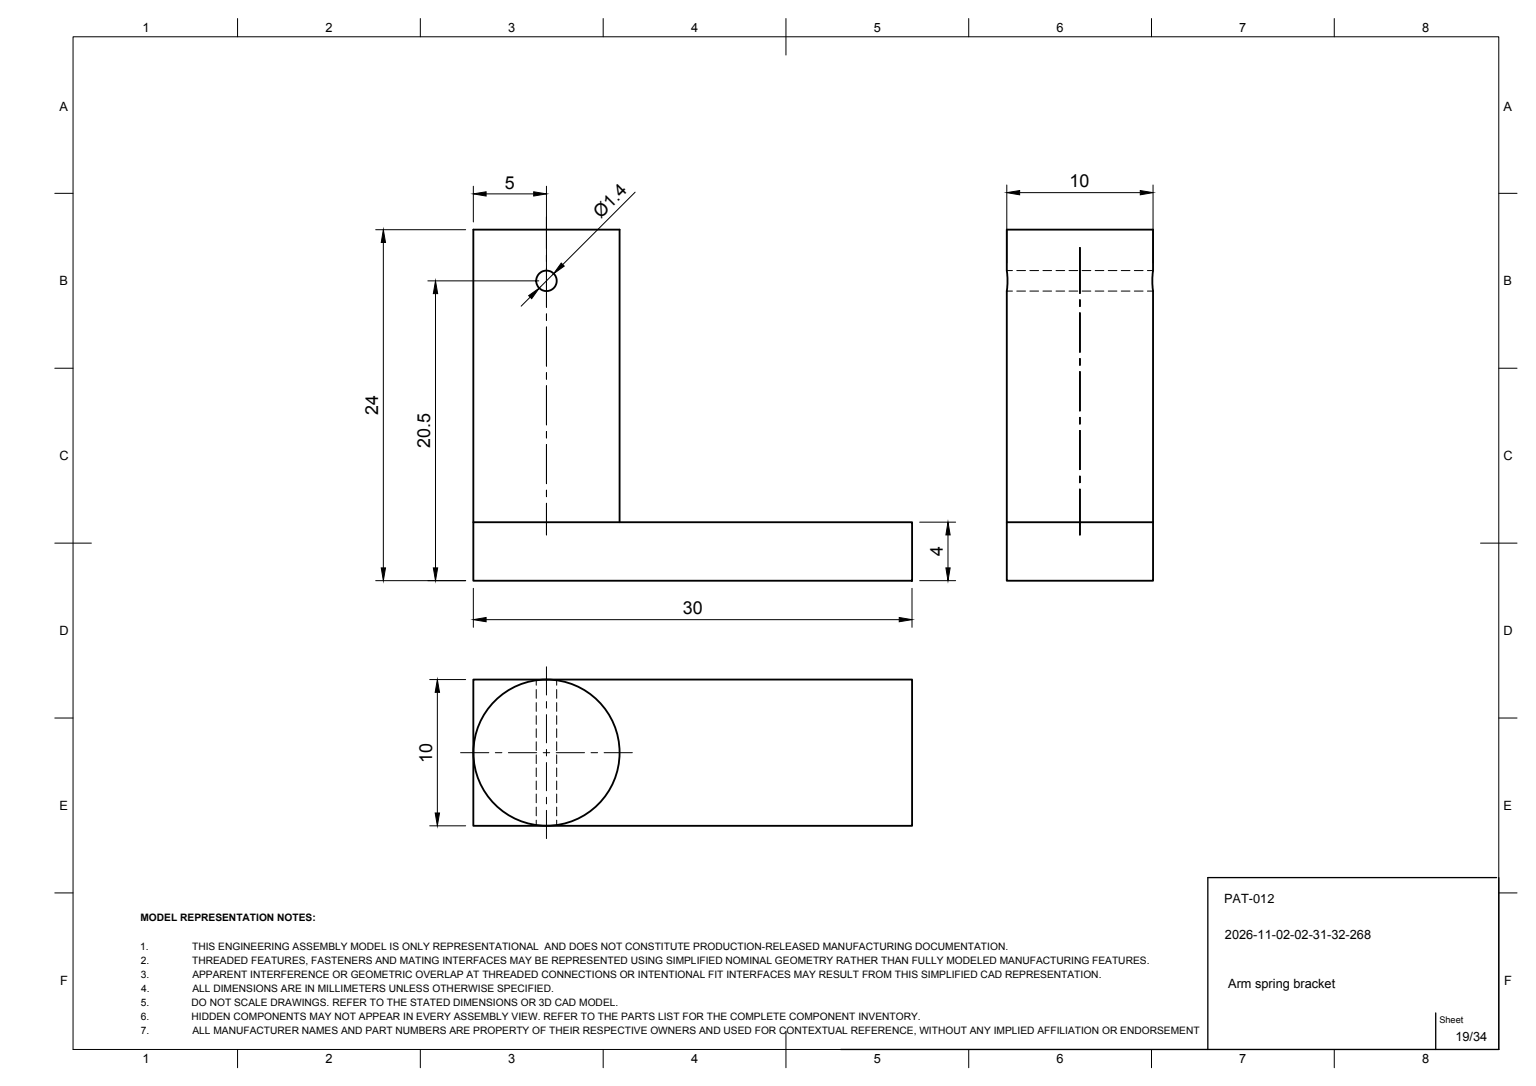
ISO-10303-21;
HEADER;
/* Generated by software containing ST-Developer
 * from STEP Tools, Inc. (www.steptools.com) 
 */

FILE_DESCRIPTION(
/* description */ ('Belt tensioner idler arm'),
/* implementation_level */ '2;1');

FILE_NAME(
/* name */ 'Arm spring bracket.step',
/* time_stamp */ '2026-10-28T03:22:15-07:00',
/* author */ (''),
/* organization */ (''),
/* preprocessor_version */ 'ST-DEVELOPER v20.2',
/* originating_system */ 'Autodesk Translation Framework v15.17.0.0',
/* authorisation */ '');

FILE_SCHEMA (('AUTOMOTIVE_DESIGN { 1 0 10303 214 3 1 1 }'));
ENDSEC;

DATA;
#10=MECHANICAL_DESIGN_GEOMETRIC_PRESENTATION_REPRESENTATION('',(#464),#12779);
#329=B_SPLINE_CURVE_WITH_KNOTS('',3,(#10963,#10964,#10965,#10966,#10967,
#10968,#10969,#10970,#10971,#10972),.UNSPECIFIED.,.F.,.F.,(4,2,2,2,4),(0.,
0.0264055269244542,0.0528110538489084,0.0792162323581899,0.105621410867471),
 .UNSPECIFIED.);
#330=B_SPLINE_CURVE_WITH_KNOTS('',3,(#10974,#10975,#10976,#10977,#10978,
#10979,#10980,#10981,#10982,#10983),.UNSPECIFIED.,.F.,.F.,(4,2,2,2,4),(0.316864232602415,
0.343269411111696,0.369674589620978,0.396080116545432,0.422485643469886),
 .UNSPECIFIED.);
#331=B_SPLINE_CURVE_WITH_KNOTS('',3,(#10984,#10985,#10986,#10987,#10988,
#10989,#10990,#10991,#10992,#10993,#10994,#10995,#10996,#10997,#10998,#10999,
#11000,#11001),.UNSPECIFIED.,.F.,.F.,(4,2,2,2,2,2,2,2,4),(0.105621410867471,
0.132026589376753,0.158431767886035,0.184837294810489,0.211242821734943,
0.237648348659397,0.264053875583851,0.290459054093133,0.316864232602415),
 .UNSPECIFIED.);
#332=B_SPLINE_CURVE_WITH_KNOTS('',3,(#11005,#11006,#11007,#11008,#11009,
#11010,#11011,#11012,#11013,#11014,#11015,#11016,#11017,#11018,#11019,#11020,
#11021,#11022,#11023,#11024,#11025,#11026,#11027,#11028,#11029,#11030),
 .UNSPECIFIED.,.F.,.F.,(4,2,2,2,2,2,2,2,2,2,2,2,4),(0.,0.0264055269244542,
0.0528110538489084,0.0792162323581899,0.105621410867471,0.132026589376753,
0.158431767886035,0.184837294810489,0.211242821734943,0.237648348659397,
0.264053875583852,0.290459054093133,0.316864232602415),.UNSPECIFIED.);
#333=B_SPLINE_CURVE_WITH_KNOTS('',3,(#11031,#11032,#11033,#11034,#11035,
#11036,#11037,#11038,#11039,#11040),.UNSPECIFIED.,.F.,.F.,(4,2,2,2,4),(0.316864232602415,
0.343269411111696,0.369674589620978,0.396080116545432,0.422485643469886),
 .UNSPECIFIED.);
#396=SHAPE_REPRESENTATION_RELATIONSHIP('SRR','None',#12943,#430);
#430=ADVANCED_BREP_SHAPE_REPRESENTATION('',(#504),#12760);
#464=STYLED_ITEM('',(#13184),#504);
#504=MANIFOLD_SOLID_BREP('Body1',#6200);
#626=FACE_BOUND('',#1480,.T.);
#756=PLANE('',#6957);
#757=PLANE('',#6958);
#758=PLANE('',#6959);
#759=PLANE('',#6960);
#760=PLANE('',#6961);
#761=PLANE('',#6962);
#762=PLANE('',#6963);
#763=PLANE('',#6964);
#764=PLANE('',#6965);
#1012=FACE_OUTER_BOUND('',#1478,.T.);
#1013=FACE_OUTER_BOUND('',#1479,.T.);
#1014=FACE_OUTER_BOUND('',#1481,.T.);
#1015=FACE_OUTER_BOUND('',#1482,.T.);
#1016=FACE_OUTER_BOUND('',#1483,.T.);
#1017=FACE_OUTER_BOUND('',#1484,.T.);
#1018=FACE_OUTER_BOUND('',#1485,.T.);
#1019=FACE_OUTER_BOUND('',#1486,.T.);
#1020=FACE_OUTER_BOUND('',#1487,.T.);
#1021=FACE_OUTER_BOUND('',#1488,.T.);
#1022=FACE_OUTER_BOUND('',#1489,.T.);
#1478=EDGE_LOOP('',(#4806,#4807,#4808,#4809,#4810,#4811,#4812));
#1479=EDGE_LOOP('',(#4813,#4814,#4815,#4816,#4817,#4818,#4819,#4820,#4821,
#4822,#4823));
#1480=EDGE_LOOP('',(#4824,#4825));
#1481=EDGE_LOOP('',(#4826));
#1482=EDGE_LOOP('',(#4827,#4828,#4829));
#1483=EDGE_LOOP('',(#4830,#4831,#4832));
#1484=EDGE_LOOP('',(#4833,#4834,#4835,#4836));
#1485=EDGE_LOOP('',(#4837,#4838,#4839,#4840,#4841));
#1486=EDGE_LOOP('',(#4842,#4843,#4844,#4845,#4846));
#1487=EDGE_LOOP('',(#4847,#4848,#4849,#4850));
#1488=EDGE_LOOP('',(#4851,#4852,#4853,#4854,#4855));
#1489=EDGE_LOOP('',(#4856,#4857,#4858,#4859));
#1889=LINE('',#11003,#2238);
#1890=LINE('',#11044,#2239);
#1891=LINE('',#11046,#2240);
#1892=LINE('',#11055,#2241);
#1893=LINE('',#11056,#2242);
#1894=LINE('',#11059,#2243);
#1895=LINE('',#11060,#2244);
#1896=LINE('',#11063,#2245);
#1897=LINE('',#11065,#2246);
#1898=LINE('',#11066,#2247);
#1899=LINE('',#11070,#2248);
#1900=LINE('',#11071,#2249);
#1901=LINE('',#11072,#2250);
#1902=LINE('',#11075,#2251);
#1903=LINE('',#11076,#2252);
#1904=LINE('',#11079,#2253);
#1905=LINE('',#11080,#2254);
#1906=LINE('',#11082,#2255);
#2238=VECTOR('',#8315,0.0700000000000003);
#2239=VECTOR('',#8320,0.5);
#2240=VECTOR('',#8321,0.5);
#2241=VECTOR('',#8332,1.);
#2242=VECTOR('',#8333,1.);
#2243=VECTOR('',#8336,1.);
#2244=VECTOR('',#8337,1.);
#2245=VECTOR('',#8340,1.);
#2246=VECTOR('',#8341,1.);
#2247=VECTOR('',#8342,1.);
#2248=VECTOR('',#8345,1.);
#2249=VECTOR('',#8346,1.);
#2250=VECTOR('',#8347,1.);
#2251=VECTOR('',#8350,1.);
#2252=VECTOR('',#8351,1.);
#2253=VECTOR('',#8354,1.);
#2254=VECTOR('',#8355,1.);
#2255=VECTOR('',#8358,1.);
#2558=CIRCLE('',#6953,0.5);
#2559=CIRCLE('',#6954,0.5);
#2560=CIRCLE('',#6955,0.5);
#2561=CIRCLE('',#6956,0.5);
#3003=VERTEX_POINT('',#10961);
#3004=VERTEX_POINT('',#10962);
#3005=VERTEX_POINT('',#10973);
#3006=VERTEX_POINT('',#11002);
#3007=VERTEX_POINT('',#11004);
#3008=VERTEX_POINT('',#11042);
#3009=VERTEX_POINT('',#11045);
#3010=VERTEX_POINT('',#11047);
#3011=VERTEX_POINT('',#11049);
#3012=VERTEX_POINT('',#11054);
#3013=VERTEX_POINT('',#11058);
#3014=VERTEX_POINT('',#11062);
#3015=VERTEX_POINT('',#11064);
#3016=VERTEX_POINT('',#11068);
#3017=VERTEX_POINT('',#11069);
#3018=VERTEX_POINT('',#11074);
#3019=VERTEX_POINT('',#11078);
#3658=EDGE_CURVE('',#3003,#3004,#329,.T.);
#3659=EDGE_CURVE('',#3005,#3003,#330,.T.);
#3660=EDGE_CURVE('',#3004,#3005,#331,.T.);
#3661=EDGE_CURVE('',#3004,#3006,#1889,.T.);
#3662=EDGE_CURVE('',#3007,#3006,#332,.T.);
#3663=EDGE_CURVE('',#3006,#3007,#333,.T.);
#3664=EDGE_CURVE('',#3008,#3008,#2558,.T.);
#3665=EDGE_CURVE('',#3008,#3004,#1890,.T.);
#3666=EDGE_CURVE('',#3005,#3009,#1891,.T.);
#3667=EDGE_CURVE('',#3010,#3009,#2559,.T.);
#3668=EDGE_CURVE('',#3011,#3010,#2560,.T.);
#3669=EDGE_CURVE('',#3009,#3011,#2561,.T.);
#3670=EDGE_CURVE('',#3011,#3012,#1892,.T.);
#3671=EDGE_CURVE('',#3012,#3009,#1893,.T.);
#3672=EDGE_CURVE('',#3010,#3013,#1894,.T.);
#3673=EDGE_CURVE('',#3013,#3011,#1895,.T.);
#3674=EDGE_CURVE('',#3009,#3014,#1896,.T.);
#3675=EDGE_CURVE('',#3014,#3015,#1897,.T.);
#3676=EDGE_CURVE('',#3015,#3010,#1898,.T.);
#3677=EDGE_CURVE('',#3016,#3017,#1899,.T.);
#3678=EDGE_CURVE('',#3017,#3012,#1900,.T.);
#3679=EDGE_CURVE('',#3016,#3013,#1901,.T.);
#3680=EDGE_CURVE('',#3018,#3016,#1902,.T.);
#3681=EDGE_CURVE('',#3018,#3015,#1903,.T.);
#3682=EDGE_CURVE('',#3019,#3018,#1904,.T.);
#3683=EDGE_CURVE('',#3019,#3014,#1905,.T.);
#3684=EDGE_CURVE('',#3017,#3019,#1906,.T.);
#4806=ORIENTED_EDGE('',*,*,#3658,.F.);
#4807=ORIENTED_EDGE('',*,*,#3659,.F.);
#4808=ORIENTED_EDGE('',*,*,#3660,.F.);
#4809=ORIENTED_EDGE('',*,*,#3661,.T.);
#4810=ORIENTED_EDGE('',*,*,#3662,.F.);
#4811=ORIENTED_EDGE('',*,*,#3663,.F.);
#4812=ORIENTED_EDGE('',*,*,#3661,.F.);
#4813=ORIENTED_EDGE('',*,*,#3664,.F.);
#4814=ORIENTED_EDGE('',*,*,#3665,.T.);
#4815=ORIENTED_EDGE('',*,*,#3660,.T.);
#4816=ORIENTED_EDGE('',*,*,#3666,.T.);
#4817=ORIENTED_EDGE('',*,*,#3667,.F.);
#4818=ORIENTED_EDGE('',*,*,#3668,.F.);
#4819=ORIENTED_EDGE('',*,*,#3669,.F.);
#4820=ORIENTED_EDGE('',*,*,#3666,.F.);
#4821=ORIENTED_EDGE('',*,*,#3659,.T.);
#4822=ORIENTED_EDGE('',*,*,#3658,.T.);
#4823=ORIENTED_EDGE('',*,*,#3665,.F.);
#4824=ORIENTED_EDGE('',*,*,#3662,.T.);
#4825=ORIENTED_EDGE('',*,*,#3663,.T.);
#4826=ORIENTED_EDGE('',*,*,#3664,.T.);
#4827=ORIENTED_EDGE('',*,*,#3669,.T.);
#4828=ORIENTED_EDGE('',*,*,#3670,.T.);
#4829=ORIENTED_EDGE('',*,*,#3671,.T.);
#4830=ORIENTED_EDGE('',*,*,#3668,.T.);
#4831=ORIENTED_EDGE('',*,*,#3672,.T.);
#4832=ORIENTED_EDGE('',*,*,#3673,.T.);
#4833=ORIENTED_EDGE('',*,*,#3667,.T.);
#4834=ORIENTED_EDGE('',*,*,#3674,.T.);
#4835=ORIENTED_EDGE('',*,*,#3675,.T.);
#4836=ORIENTED_EDGE('',*,*,#3676,.T.);
#4837=ORIENTED_EDGE('',*,*,#3677,.T.);
#4838=ORIENTED_EDGE('',*,*,#3678,.T.);
#4839=ORIENTED_EDGE('',*,*,#3670,.F.);
#4840=ORIENTED_EDGE('',*,*,#3673,.F.);
#4841=ORIENTED_EDGE('',*,*,#3679,.F.);
#4842=ORIENTED_EDGE('',*,*,#3680,.T.);
#4843=ORIENTED_EDGE('',*,*,#3679,.T.);
#4844=ORIENTED_EDGE('',*,*,#3672,.F.);
#4845=ORIENTED_EDGE('',*,*,#3676,.F.);
#4846=ORIENTED_EDGE('',*,*,#3681,.F.);
#4847=ORIENTED_EDGE('',*,*,#3682,.T.);
#4848=ORIENTED_EDGE('',*,*,#3681,.T.);
#4849=ORIENTED_EDGE('',*,*,#3675,.F.);
#4850=ORIENTED_EDGE('',*,*,#3683,.F.);
#4851=ORIENTED_EDGE('',*,*,#3684,.T.);
#4852=ORIENTED_EDGE('',*,*,#3683,.T.);
#4853=ORIENTED_EDGE('',*,*,#3674,.F.);
#4854=ORIENTED_EDGE('',*,*,#3671,.F.);
#4855=ORIENTED_EDGE('',*,*,#3678,.F.);
#4856=ORIENTED_EDGE('',*,*,#3684,.F.);
#4857=ORIENTED_EDGE('',*,*,#3677,.F.);
#4858=ORIENTED_EDGE('',*,*,#3680,.F.);
#4859=ORIENTED_EDGE('',*,*,#3682,.F.);
#5732=CYLINDRICAL_SURFACE('',#6951,0.0700000000000003);
#5733=CYLINDRICAL_SURFACE('',#6952,0.5);
#5989=ADVANCED_FACE('',(#1012),#5732,.F.);
#5990=ADVANCED_FACE('',(#1013,#626),#5733,.T.);
#5991=ADVANCED_FACE('',(#1014),#756,.T.);
#5992=ADVANCED_FACE('',(#1015),#757,.T.);
#5993=ADVANCED_FACE('',(#1016),#758,.T.);
#5994=ADVANCED_FACE('',(#1017),#759,.T.);
#5995=ADVANCED_FACE('',(#1018),#760,.T.);
#5996=ADVANCED_FACE('',(#1019),#761,.T.);
#5997=ADVANCED_FACE('',(#1020),#762,.T.);
#5998=ADVANCED_FACE('',(#1021),#763,.T.);
#5999=ADVANCED_FACE('',(#1022),#764,.F.);
#6200=CLOSED_SHELL('',(#5989,#5990,#5991,#5992,#5993,#5994,#5995,#5996,
#5997,#5998,#5999));
#6950=AXIS2_PLACEMENT_3D('',#10959,#8311,#8312);
#6951=AXIS2_PLACEMENT_3D('',#10960,#8313,#8314);
#6952=AXIS2_PLACEMENT_3D('',#11041,#8316,#8317);
#6953=AXIS2_PLACEMENT_3D('',#11043,#8318,#8319);
#6954=AXIS2_PLACEMENT_3D('',#11048,#8322,#8323);
#6955=AXIS2_PLACEMENT_3D('',#11050,#8324,#8325);
#6956=AXIS2_PLACEMENT_3D('',#11051,#8326,#8327);
#6957=AXIS2_PLACEMENT_3D('',#11052,#8328,#8329);
#6958=AXIS2_PLACEMENT_3D('',#11053,#8330,#8331);
#6959=AXIS2_PLACEMENT_3D('',#11057,#8334,#8335);
#6960=AXIS2_PLACEMENT_3D('',#11061,#8338,#8339);
#6961=AXIS2_PLACEMENT_3D('',#11067,#8343,#8344);
#6962=AXIS2_PLACEMENT_3D('',#11073,#8348,#8349);
#6963=AXIS2_PLACEMENT_3D('',#11077,#8352,#8353);
#6964=AXIS2_PLACEMENT_3D('',#11081,#8356,#8357);
#6965=AXIS2_PLACEMENT_3D('',#11083,#8359,#8360);
#8311=DIRECTION('axis',(0.,0.,1.));
#8312=DIRECTION('refdir',(1.,0.,0.));
#8313=DIRECTION('center_axis',(1.,0.,0.));
#8314=DIRECTION('ref_axis',(0.,0.,-1.));
#8315=DIRECTION('',(1.,0.,0.));
#8316=DIRECTION('center_axis',(0.,0.,1.));
#8317=DIRECTION('ref_axis',(1.,0.,0.));
#8318=DIRECTION('center_axis',(0.,0.,1.));
#8319=DIRECTION('ref_axis',(1.,0.,0.));
#8320=DIRECTION('',(0.,0.,-1.));
#8321=DIRECTION('',(0.,0.,-1.));
#8322=DIRECTION('center_axis',(0.,0.,-1.));
#8323=DIRECTION('ref_axis',(1.,0.,0.));
#8324=DIRECTION('center_axis',(0.,0.,-1.));
#8325=DIRECTION('ref_axis',(1.,0.,0.));
#8326=DIRECTION('center_axis',(0.,0.,-1.));
#8327=DIRECTION('ref_axis',(1.,0.,0.));
#8328=DIRECTION('center_axis',(0.,0.,1.));
#8329=DIRECTION('ref_axis',(1.,0.,0.));
#8330=DIRECTION('center_axis',(0.,0.,1.));
#8331=DIRECTION('ref_axis',(1.,0.,0.));
#8332=DIRECTION('',(-1.,0.,0.));
#8333=DIRECTION('',(0.,-1.,0.));
#8334=DIRECTION('center_axis',(0.,0.,1.));
#8335=DIRECTION('ref_axis',(1.,0.,0.));
#8336=DIRECTION('',(0.,1.,0.));
#8337=DIRECTION('',(-1.,0.,0.));
#8338=DIRECTION('center_axis',(0.,0.,1.));
#8339=DIRECTION('ref_axis',(1.,0.,0.));
#8340=DIRECTION('',(0.,-1.,0.));
#8341=DIRECTION('',(1.,0.,0.));
#8342=DIRECTION('',(0.,1.,0.));
#8343=DIRECTION('center_axis',(0.,1.,0.));
#8344=DIRECTION('ref_axis',(-1.,0.,0.));
#8345=DIRECTION('',(-1.,0.,0.));
#8346=DIRECTION('',(0.,0.,1.));
#8347=DIRECTION('',(0.,0.,1.));
#8348=DIRECTION('center_axis',(1.,0.,0.));
#8349=DIRECTION('ref_axis',(0.,1.,0.));
#8350=DIRECTION('',(0.,1.,0.));
#8351=DIRECTION('',(0.,0.,1.));
#8352=DIRECTION('center_axis',(0.,-1.,0.));
#8353=DIRECTION('ref_axis',(1.,0.,0.));
#8354=DIRECTION('',(1.,0.,0.));
#8355=DIRECTION('',(0.,0.,1.));
#8356=DIRECTION('center_axis',(-1.,0.,0.));
#8357=DIRECTION('ref_axis',(0.,-1.,0.));
#8358=DIRECTION('',(0.,-1.,0.));
#8359=DIRECTION('center_axis',(0.,0.,1.));
#8360=DIRECTION('ref_axis',(1.,0.,0.));
#10959=CARTESIAN_POINT('',(0.,0.,0.));
#10960=CARTESIAN_POINT('Origin',(2.4,2.5,8.05));
#10961=CARTESIAN_POINT('',(2.50492424822054,2.57,8.05));
#10962=CARTESIAN_POINT('',(2.5,2.5,8.12));
#10963=CARTESIAN_POINT('Ctrl Pts',(2.50492424822054,2.57,8.05));
#10964=CARTESIAN_POINT('Ctrl Pts',(2.50492424822054,2.57,8.05880184230815));
#10965=CARTESIAN_POINT('Ctrl Pts',(2.50466528015196,2.56823857908987,8.06818235803024));
#10966=CARTESIAN_POINT('Ctrl Pts',(2.50373308905894,2.56109125434544,8.08542542296838));
#10967=CARTESIAN_POINT('Ctrl Pts',(2.50307367614139,2.5557059746568,8.09328897470932));
#10968=CARTESIAN_POINT('Ctrl Pts',(2.50183839619558,2.54328905662912,8.10570589273699));
#10969=CARTESIAN_POINT('Ctrl Pts',(2.50118181447624,2.53542546943526,8.11109123666712));
#10970=CARTESIAN_POINT('Ctrl Pts',(2.50025611494785,2.51818228380197,8.11823860827541));
#10971=CARTESIAN_POINT('Ctrl Pts',(2.5,2.50880172616976,8.12));
#10972=CARTESIAN_POINT('Ctrl Pts',(2.5,2.5,8.12));
#10973=CARTESIAN_POINT('',(2.5,2.5,7.98));
#10974=CARTESIAN_POINT('Ctrl Pts',(2.5,2.5,7.98));
#10975=CARTESIAN_POINT('Ctrl Pts',(2.5,2.50880172616976,7.98));
#10976=CARTESIAN_POINT('Ctrl Pts',(2.50025611494785,2.51818228380197,7.98176139172459));
#10977=CARTESIAN_POINT('Ctrl Pts',(2.50118181447624,2.53542546943525,7.98890876333288));
#10978=CARTESIAN_POINT('Ctrl Pts',(2.50183839619558,2.54328905662912,7.99429410726301));
#10979=CARTESIAN_POINT('Ctrl Pts',(2.50307367614139,2.5557059746568,8.00671102529068));
#10980=CARTESIAN_POINT('Ctrl Pts',(2.50373308905894,2.56109125434544,8.01457457703162));
#10981=CARTESIAN_POINT('Ctrl Pts',(2.50466528015196,2.56823857908987,8.03181764196976));
#10982=CARTESIAN_POINT('Ctrl Pts',(2.50492424822054,2.57,8.04119815769185));
#10983=CARTESIAN_POINT('Ctrl Pts',(2.50492424822054,2.57,8.05));
#10984=CARTESIAN_POINT('Ctrl Pts',(2.5,2.5,8.12));
#10985=CARTESIAN_POINT('Ctrl Pts',(2.5,2.49119827383024,8.12));
#10986=CARTESIAN_POINT('Ctrl Pts',(2.50025611494785,2.48181771619803,8.11823860827541));
#10987=CARTESIAN_POINT('Ctrl Pts',(2.50118181447624,2.46457453056474,8.11109123666712));
#10988=CARTESIAN_POINT('Ctrl Pts',(2.50183839619558,2.45671094337088,8.10570589273699));
#10989=CARTESIAN_POINT('Ctrl Pts',(2.50307367614139,2.4442940253432,8.09328897470932));
#10990=CARTESIAN_POINT('Ctrl Pts',(2.50373308905894,2.43890874565455,8.08542542296837));
#10991=CARTESIAN_POINT('Ctrl Pts',(2.50466528015196,2.43176142091013,8.06818235803023));
#10992=CARTESIAN_POINT('Ctrl Pts',(2.50492424822054,2.43,8.05880184230815));
#10993=CARTESIAN_POINT('Ctrl Pts',(2.50492424822054,2.43,8.04119815769185));
#10994=CARTESIAN_POINT('Ctrl Pts',(2.50466528015196,2.43176142091014,8.03181764196976));
#10995=CARTESIAN_POINT('Ctrl Pts',(2.50373308905894,2.43890874565456,8.01457457703162));
#10996=CARTESIAN_POINT('Ctrl Pts',(2.50307367614139,2.4442940253432,8.00671102529068));
#10997=CARTESIAN_POINT('Ctrl Pts',(2.50183839619558,2.45671094337088,7.99429410726301));
#10998=CARTESIAN_POINT('Ctrl Pts',(2.50118181447624,2.46457453056474,7.98890876333288));
#10999=CARTESIAN_POINT('Ctrl Pts',(2.50025611494785,2.48181771619803,7.98176139172459));
#11000=CARTESIAN_POINT('Ctrl Pts',(2.5,2.49119827383024,7.98));
#11001=CARTESIAN_POINT('Ctrl Pts',(2.5,2.5,7.98));
#11002=CARTESIAN_POINT('',(3.5,2.5,8.12));
#11003=CARTESIAN_POINT('',(2.4,2.5,8.12));
#11004=CARTESIAN_POINT('',(3.49507575177946,2.57,8.05));
#11005=CARTESIAN_POINT('Ctrl Pts',(3.49507575177946,2.57,8.05));
#11006=CARTESIAN_POINT('Ctrl Pts',(3.49507575177946,2.57,8.04119815769185));
#11007=CARTESIAN_POINT('Ctrl Pts',(3.49533471984804,2.56823857908987,8.03181764196976));
#11008=CARTESIAN_POINT('Ctrl Pts',(3.49626691094106,2.56109125434544,8.01457457703162));
#11009=CARTESIAN_POINT('Ctrl Pts',(3.49692632385861,2.5557059746568,8.00671102529068));
#11010=CARTESIAN_POINT('Ctrl Pts',(3.49816160380442,2.54328905662912,7.99429410726301));
#11011=CARTESIAN_POINT('Ctrl Pts',(3.49881818552376,2.53542546943526,7.98890876333288));
#11012=CARTESIAN_POINT('Ctrl Pts',(3.49974388505215,2.51818228380197,7.98176139172459));
#11013=CARTESIAN_POINT('Ctrl Pts',(3.5,2.50880172616976,7.98));
#11014=CARTESIAN_POINT('Ctrl Pts',(3.5,2.49119827383024,7.98));
#11015=CARTESIAN_POINT('Ctrl Pts',(3.49974388505215,2.48181771619803,7.98176139172459));
#11016=CARTESIAN_POINT('Ctrl Pts',(3.49881818552376,2.46457453056474,7.98890876333288));
#11017=CARTESIAN_POINT('Ctrl Pts',(3.49816160380442,2.45671094337088,7.99429410726301));
#11018=CARTESIAN_POINT('Ctrl Pts',(3.49692632385861,2.4442940253432,8.00671102529068));
#11019=CARTESIAN_POINT('Ctrl Pts',(3.49626691094106,2.43890874565456,8.01457457703162));
#11020=CARTESIAN_POINT('Ctrl Pts',(3.49533471984804,2.43176142091013,8.03181764196976));
#11021=CARTESIAN_POINT('Ctrl Pts',(3.49507575177946,2.43,8.04119815769185));
#11022=CARTESIAN_POINT('Ctrl Pts',(3.49507575177946,2.43,8.05880184230815));
#11023=CARTESIAN_POINT('Ctrl Pts',(3.49533471984804,2.43176142091013,8.06818235803024));
#11024=CARTESIAN_POINT('Ctrl Pts',(3.49626691094106,2.43890874565456,8.08542542296838));
#11025=CARTESIAN_POINT('Ctrl Pts',(3.49692632385861,2.4442940253432,8.09328897470932));
#11026=CARTESIAN_POINT('Ctrl Pts',(3.49816160380442,2.45671094337088,8.10570589273699));
#11027=CARTESIAN_POINT('Ctrl Pts',(3.49881818552376,2.46457453056474,8.11109123666712));
#11028=CARTESIAN_POINT('Ctrl Pts',(3.49974388505215,2.48181771619803,8.11823860827541));
#11029=CARTESIAN_POINT('Ctrl Pts',(3.5,2.49119827383024,8.12));
#11030=CARTESIAN_POINT('Ctrl Pts',(3.5,2.5,8.12));
#11031=CARTESIAN_POINT('Ctrl Pts',(3.5,2.5,8.12));
#11032=CARTESIAN_POINT('Ctrl Pts',(3.5,2.50880172616976,8.12));
#11033=CARTESIAN_POINT('Ctrl Pts',(3.49974388505215,2.51818228380197,8.11823860827541));
#11034=CARTESIAN_POINT('Ctrl Pts',(3.49881818552376,2.53542546943526,8.11109123666712));
#11035=CARTESIAN_POINT('Ctrl Pts',(3.49816160380442,2.54328905662912,8.10570589273699));
#11036=CARTESIAN_POINT('Ctrl Pts',(3.49692632385861,2.5557059746568,8.09328897470932));
#11037=CARTESIAN_POINT('Ctrl Pts',(3.49626691094106,2.56109125434544,8.08542542296838));
#11038=CARTESIAN_POINT('Ctrl Pts',(3.49533471984804,2.56823857908987,8.06818235803024));
#11039=CARTESIAN_POINT('Ctrl Pts',(3.49507575177946,2.57,8.05880184230815));
#11040=CARTESIAN_POINT('Ctrl Pts',(3.49507575177946,2.57,8.05));
#11041=CARTESIAN_POINT('Origin',(3.,2.5,6.4));
#11042=CARTESIAN_POINT('',(2.5,2.5,8.4));
#11043=CARTESIAN_POINT('Origin',(3.,2.5,8.4));
#11044=CARTESIAN_POINT('',(2.5,2.5,6.4));
#11045=CARTESIAN_POINT('',(2.5,2.5,6.4));
#11046=CARTESIAN_POINT('',(2.5,2.5,6.4));
#11047=CARTESIAN_POINT('',(3.5,2.5,6.4));
#11048=CARTESIAN_POINT('Origin',(3.,2.5,6.4));
#11049=CARTESIAN_POINT('',(3.,3.,6.4));
#11050=CARTESIAN_POINT('Origin',(3.,2.5,6.4));
#11051=CARTESIAN_POINT('Origin',(3.,2.5,6.4));
#11052=CARTESIAN_POINT('Origin',(3.,2.5,8.4));
#11053=CARTESIAN_POINT('Origin',(3.,1.5,6.4));
#11054=CARTESIAN_POINT('',(2.5,3.,6.4));
#11055=CARTESIAN_POINT('',(3.5,3.,6.4));
#11056=CARTESIAN_POINT('',(2.5,3.,6.4));
#11057=CARTESIAN_POINT('Origin',(3.,1.5,6.4));
#11058=CARTESIAN_POINT('',(3.5,3.,6.4));
#11059=CARTESIAN_POINT('',(3.5,0.,6.4));
#11060=CARTESIAN_POINT('',(3.5,3.,6.4));
#11061=CARTESIAN_POINT('Origin',(3.,1.5,6.4));
#11062=CARTESIAN_POINT('',(2.5,0.,6.4));
#11063=CARTESIAN_POINT('',(2.5,3.,6.4));
#11064=CARTESIAN_POINT('',(3.5,0.,6.4));
#11065=CARTESIAN_POINT('',(2.5,0.,6.4));
#11066=CARTESIAN_POINT('',(3.5,0.,6.4));
#11067=CARTESIAN_POINT('Origin',(3.5,3.,6.));
#11068=CARTESIAN_POINT('',(3.5,3.,6.));
#11069=CARTESIAN_POINT('',(2.5,3.,6.));
#11070=CARTESIAN_POINT('',(3.5,3.,6.));
#11071=CARTESIAN_POINT('',(2.5,3.,6.));
#11072=CARTESIAN_POINT('',(3.5,3.,6.));
#11073=CARTESIAN_POINT('Origin',(3.5,0.,6.));
#11074=CARTESIAN_POINT('',(3.5,0.,6.));
#11075=CARTESIAN_POINT('',(3.5,0.,6.));
#11076=CARTESIAN_POINT('',(3.5,0.,6.));
#11077=CARTESIAN_POINT('Origin',(2.5,0.,6.));
#11078=CARTESIAN_POINT('',(2.5,0.,6.));
#11079=CARTESIAN_POINT('',(2.5,0.,6.));
#11080=CARTESIAN_POINT('',(2.5,0.,6.));
#11081=CARTESIAN_POINT('Origin',(2.5,3.,6.));
#11082=CARTESIAN_POINT('',(2.5,3.,6.));
#11083=CARTESIAN_POINT('Origin',(3.,1.5,6.));
#12720=UNCERTAINTY_MEASURE_WITH_UNIT(LENGTH_MEASURE(0.001),#12780,
'DISTANCE_ACCURACY_VALUE',
'Maximum model space distance between geometric entities at asserted c
onnectivities');
#12739=UNCERTAINTY_MEASURE_WITH_UNIT(LENGTH_MEASURE(0.001),#12780,
'DISTANCE_ACCURACY_VALUE',
'Maximum model space distance between geometric entities at asserted c
onnectivities');
#12760=(
GEOMETRIC_REPRESENTATION_CONTEXT(3)
GLOBAL_UNCERTAINTY_ASSIGNED_CONTEXT((#12720))
GLOBAL_UNIT_ASSIGNED_CONTEXT((#12780,#12782,#12783))
REPRESENTATION_CONTEXT('','3D')
);
#12779=(
GEOMETRIC_REPRESENTATION_CONTEXT(3)
GLOBAL_UNCERTAINTY_ASSIGNED_CONTEXT((#12739))
GLOBAL_UNIT_ASSIGNED_CONTEXT((#12780,#12782,#12783))
REPRESENTATION_CONTEXT('','3D')
);
#12780=(
LENGTH_UNIT()
NAMED_UNIT(*)
SI_UNIT(.CENTI.,.METRE.)
);
#12782=(
NAMED_UNIT(*)
PLANE_ANGLE_UNIT()
SI_UNIT($,.RADIAN.)
);
#12783=(
NAMED_UNIT(*)
SI_UNIT($,.STERADIAN.)
SOLID_ANGLE_UNIT()
);
#12804=SHAPE_DEFINITION_REPRESENTATION(#12843,#12943);
#12843=PRODUCT_DEFINITION_SHAPE('',$,#12983);
#12943=SHAPE_REPRESENTATION('',(#6950),#12760);
#12962=PRODUCT_DEFINITION_CONTEXT('part definition',#13081,'design');
#12983=PRODUCT_DEFINITION('Arm spring bracket','Arm spring bracket',#13022,
#12962);
#13022=PRODUCT_DEFINITION_FORMATION('',$,#13103);
#13081=APPLICATION_CONTEXT(
'Core Data for Automotive Mechanical Design Process');
#13082=PRODUCT_CONTEXT('part definition',#13081,'mechanical');
#13103=PRODUCT('Arm spring bracket','Arm spring bracket',
'Arm spring bracket',(#13082));
#13178=COLOUR_RGB('Grey',0.48,0.52,0.57);
#13179=FILL_AREA_STYLE_COLOUR('',#13178);
#13180=FILL_AREA_STYLE('',(#13179));
#13181=SURFACE_STYLE_FILL_AREA(#13180);
#13182=SURFACE_SIDE_STYLE('',(#13181));
#13183=SURFACE_STYLE_USAGE(.BOTH.,#13182);
#13184=PRESENTATION_STYLE_ASSIGNMENT((#13183));
ENDSEC;
END-ISO-10303-21;
